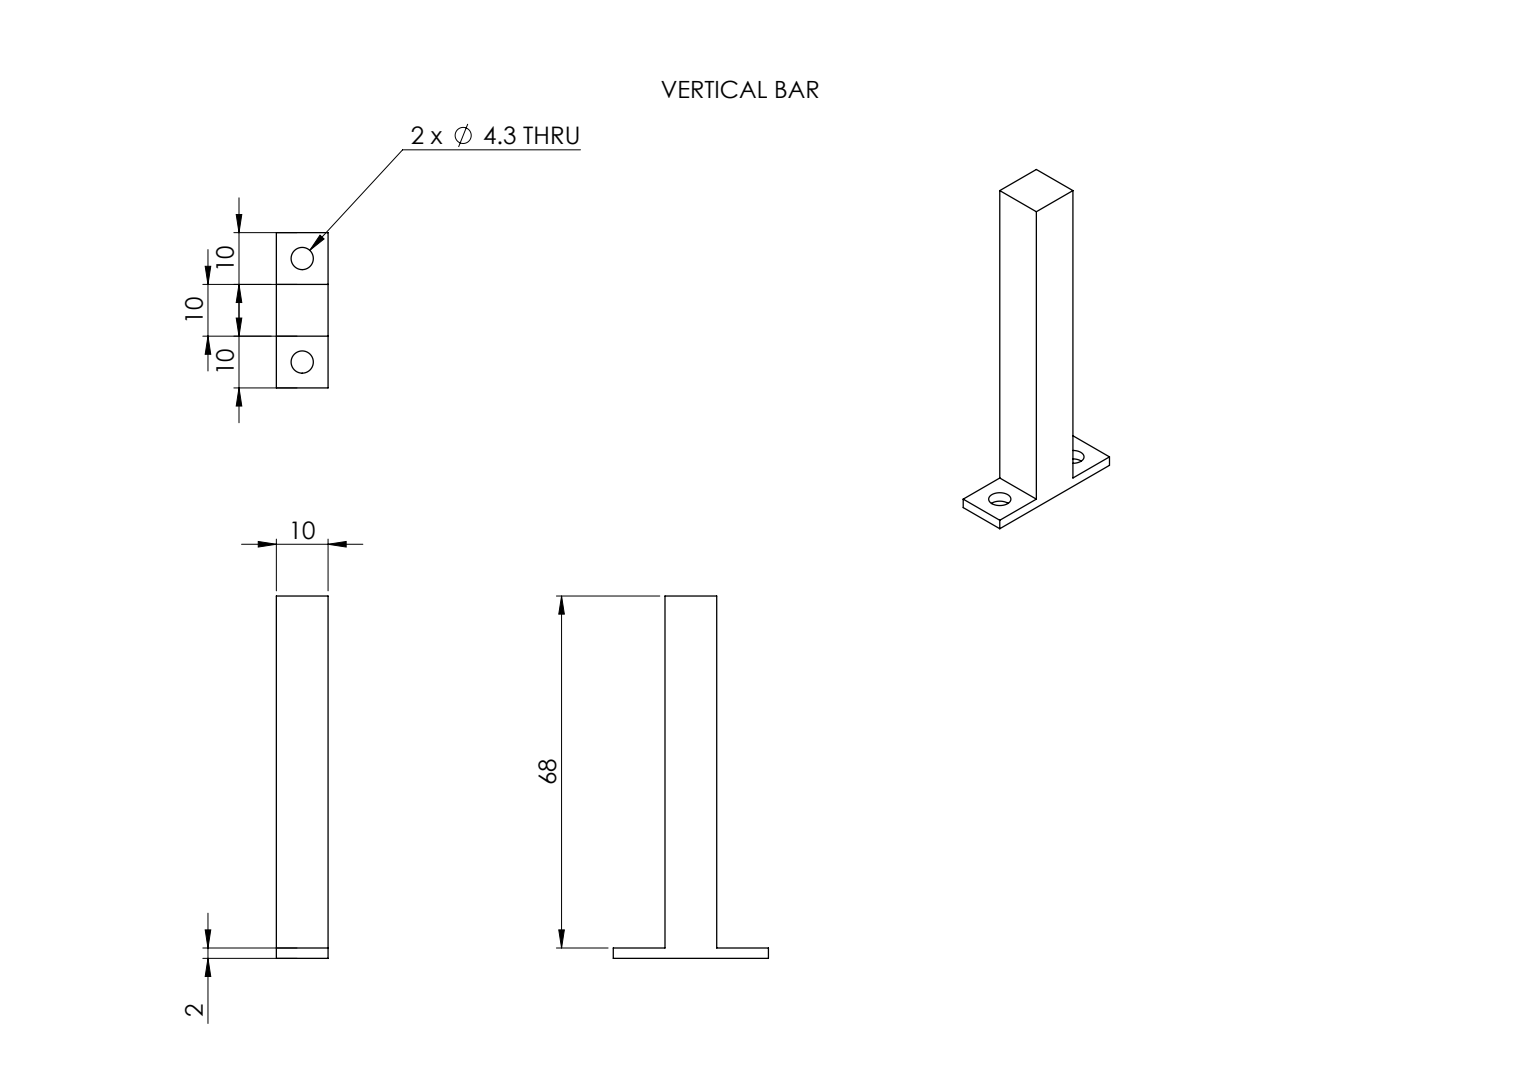
ISO-10303-21;
HEADER;
FILE_DESCRIPTION (('STEP AP214'),
    '1' );
FILE_NAME ('vertical bar^MAS-192.step',
    '2026-10-24T04:45:50',
    ( '' ),
    ( '' ),
    'SwSTEP 2.0',
    'SolidWorks 2026',
    '' );
FILE_SCHEMA (( 'AUTOMOTIVE_DESIGN' ));
ENDSEC;

DATA;
#7=( GEOMETRIC_REPRESENTATION_CONTEXT ( 3 ) GLOBAL_UNCERTAINTY_ASSIGNED_CONTEXT ( ( #487 ) ) GLOBAL_UNIT_ASSIGNED_CONTEXT ( ( #3000, #1213, #165 ) ) REPRESENTATION_CONTEXT ( 'NONE', 'WORKASPACE' ) );
#18=CARTESIAN_POINT ( 'NONE',  ( -49.99999999999999289, 52.00000000000000711, -14.99999999999999645 ) ) ;
#30=CARTESIAN_POINT ( 'NONE',  ( -45.00000000000000000, 52.00000000000000711, -7.849999999999996092 ) ) ;
#40=AXIS2_PLACEMENT_3D ( 'NONE', #1566, #1549, #2083 ) ;
#49=AXIS2_PLACEMENT_3D ( 'NONE', #2635, #3135, #2647 ) ;
#59=VECTOR ( 'NONE', #1910, 1000.000000000000000 ) ;
#68=DIRECTION ( 'NONE',  ( -1.000000000000000000, -0.000000000000000000, -0.000000000000000000 ) ) ;
#69=CARTESIAN_POINT ( 'NONE',  ( -45.00000000000000000, 52.00000000000000711, -9.999999999999994671 ) ) ;
#91=ORIENTED_EDGE ( 'NONE', *, *, #1822, .T. ) ;
#99=DIRECTION ( 'NONE',  ( 0.000000000000000000, -1.000000000000000000, -0.000000000000000000 ) ) ;
#130=LINE ( 'NONE', #2502, #3267 ) ;
#137=EDGE_CURVE ( 'NONE', #1848, #2577, #1400, .T. ) ;
#143=CARTESIAN_POINT ( 'NONE',  ( -49.99999999999998579, 50.00000000000000000, 15.00000000000000888 ) ) ;
#165=( NAMED_UNIT ( * ) SI_UNIT ( $, .STERADIAN. ) SOLID_ANGLE_UNIT ( ) );
#174=CARTESIAN_POINT ( 'NONE',  ( -44.99999999999999289, 52.00000000000000711, 10.00000000000000533 ) ) ;
#177=ADVANCED_FACE ( 'NONE', ( #782 ), #2573, .F. ) ;
#181=EDGE_CURVE ( 'NONE', #2222, #1240, #233, .T. ) ;
#189=DIRECTION ( 'NONE',  ( 0.000000000000000000, 0.000000000000000000, 1.000000000000000000 ) ) ;
#190=VERTEX_POINT ( 'NONE', #1045 ) ;
#194=CARTESIAN_POINT ( 'NONE',  ( -49.99999999999999289, 52.00000000000000711, -4.999999999999995559 ) ) ;
#197=DIRECTION ( 'NONE',  ( -0.000000000000000000, 1.000000000000000000, -0.000000000000000000 ) ) ;
#198=CARTESIAN_POINT ( 'NONE',  ( -50.00000000000000000, 120.0000000000000142, 5.000000000000004441 ) ) ;
#214=ORIENTED_EDGE ( 'NONE', *, *, #2529, .F. ) ;
#217=CARTESIAN_POINT ( 'NONE',  ( -45.00000000000000000, 50.00000000000000000, -9.999999999999994671 ) ) ;
#224=ORIENTED_EDGE ( 'NONE', *, *, #1328, .F. ) ;
#229=VERTEX_POINT ( 'NONE', #2063 ) ;
#233=LINE ( 'NONE', #18, #635 ) ;
#235=PRODUCT ( 'vertical bar^MAS-192', 'vertical bar^MAS-192', '', ( #1405 ) ) ;
#239=DIRECTION ( 'NONE',  ( 1.000000000000000000, 0.000000000000000000, 0.000000000000000000 ) ) ;
#256=PLANE ( 'NONE',  #3270 ) ;
#259=EDGE_CURVE ( 'NONE', #2577, #1848, #1348, .T. ) ;
#285=ORIENTED_EDGE ( 'NONE', *, *, #1596, .F. ) ;
#299=ORIENTED_EDGE ( 'NONE', *, *, #1600, .T. ) ;
#311=FACE_OUTER_BOUND ( 'NONE', #2869, .T. ) ;
#313=ORIENTED_EDGE ( 'NONE', *, *, #934, .T. ) ;
#315=ADVANCED_BREP_SHAPE_REPRESENTATION ( '', ( #2820, #3111 ), #7 ) ;
#316=LINE ( 'NONE', #2146, #2603 ) ;
#318=CIRCLE ( 'NONE', #2498, 2.149999999999999023 ) ;
#326=ORIENTED_EDGE ( 'NONE', *, *, #789, .T. ) ;
#327=EDGE_LOOP ( 'NONE', ( #1272, #3114, #2142, #1931 ) ) ;
#328=FACE_OUTER_BOUND ( 'NONE', #327, .T. ) ;
#336=DIRECTION ( 'NONE',  ( 6.938893903907228378E-16, 0.000000000000000000, 1.000000000000000000 ) ) ;
#344=CARTESIAN_POINT ( 'NONE',  ( -49.99999999999999289, 52.00000000000000711, -14.99999999999999645 ) ) ;
#353=FACE_OUTER_BOUND ( 'NONE', #793, .T. ) ;
#355=EDGE_LOOP ( 'NONE', ( #2017, #2646, #2374, #1630 ) ) ;
#356=LINE ( 'NONE', #823, #1685 ) ;
#358=ORIENTED_EDGE ( 'NONE', *, *, #750, .T. ) ;
#359=CARTESIAN_POINT ( 'NONE',  ( -44.99999999999999289, 50.00000000000000000, 10.00000000000000533 ) ) ;
#361=VERTEX_POINT ( 'NONE', #3180 ) ;
#373=AXIS2_PLACEMENT_3D ( 'NONE', #3007, #3300, #957 ) ;
#392=EDGE_CURVE ( 'NONE', #2543, #2273, #1858, .T. ) ;
#399=DIRECTION ( 'NONE',  ( -0.000000000000000000, 1.000000000000000000, -0.000000000000000000 ) ) ;
#404=FILL_AREA_STYLE_COLOUR ( '', #874 ) ;
#430=LINE ( 'NONE', #1761, #2389 ) ;
#439=( NAMED_UNIT ( * ) PLANE_ANGLE_UNIT ( ) SI_UNIT ( $, .RADIAN. ) );
#447=( LENGTH_UNIT ( ) NAMED_UNIT ( * ) SI_UNIT ( .MILLI., .METRE. ) );
#449=LINE ( 'NONE', #959, #1301 ) ;
#465=ORIENTED_EDGE ( 'NONE', *, *, #2720, .F. ) ;
#471=DIRECTION ( 'NONE',  ( -0.000000000000000000, 1.000000000000000000, -0.000000000000000000 ) ) ;
#476=ORIENTED_EDGE ( 'NONE', *, *, #2240, .T. ) ;
#481=DIRECTION ( 'NONE',  ( 0.000000000000000000, -0.000000000000000000, -1.000000000000000000 ) ) ;
#487=UNCERTAINTY_MEASURE_WITH_UNIT (LENGTH_MEASURE( 1.000000000000000082E-05 ), #3000, 'distance_accuracy_value', 'NONE');
#491=DIRECTION ( 'NONE',  ( -0.000000000000000000, -1.000000000000000000, -0.000000000000000000 ) ) ;
#493=LINE ( 'NONE', #2046, #2452 ) ;
#496=EDGE_CURVE ( 'NONE', #1994, #2222, #130, .T. ) ;
#500=LINE ( 'NONE', #2579, #1737 ) ;
#517=DIRECTION ( 'NONE',  ( -0.000000000000000000, 1.000000000000000000, -0.000000000000000000 ) ) ;
#524=( NAMED_UNIT ( * ) SI_UNIT ( $, .STERADIAN. ) SOLID_ANGLE_UNIT ( ) );
#526=ORIENTED_EDGE ( 'NONE', *, *, #934, .F. ) ;
#529=VECTOR ( 'NONE', #491, 1000.000000000000000 ) ;
#534=VECTOR ( 'NONE', #1624, 1000.000000000000000 ) ;
#538=ORIENTED_EDGE ( 'NONE', *, *, #496, .F. ) ;
#539=DIRECTION ( 'NONE',  ( 0.000000000000000000, -1.000000000000000000, 0.000000000000000000 ) ) ;
#542=AXIS2_PLACEMENT_3D ( 'NONE', #1565, #1586, #1044 ) ;
#558=DIRECTION ( 'NONE',  ( -1.000000000000000000, 0.000000000000000000, 6.938893903907232322E-16 ) ) ;
#574=DIRECTION ( 'NONE',  ( 0.000000000000000000, 0.000000000000000000, 1.000000000000000000 ) ) ;
#580=CARTESIAN_POINT ( 'NONE',  ( -45.00000000000000000, 50.00000000000000000, -7.849999999999996092 ) ) ;
#585=CARTESIAN_POINT ( 'NONE',  ( -44.99999999999999289, 50.00000000000000000, 10.00000000000000533 ) ) ;
#608=VERTEX_POINT ( 'NONE', #2329 ) ;
#610=DIRECTION ( 'NONE',  ( 6.938893903907228378E-16, 0.000000000000000000, -1.000000000000000000 ) ) ;
#614=PLANE ( 'NONE',  #3101 ) ;
#619=EDGE_CURVE ( 'NONE', #1240, #2273, #742, .T. ) ;
#624=VERTEX_POINT ( 'NONE', #2550 ) ;
#635=VECTOR ( 'NONE', #1006, 1000.000000000000000 ) ;
#643=VECTOR ( 'NONE', #2325, 1000.000000000000000 ) ;
#652=LINE ( 'NONE', #1697, #534 ) ;
#667=ORIENTED_EDGE ( 'NONE', *, *, #2408, .F. ) ;
#677=PLANE ( 'NONE',  #2180 ) ;
#682=ORIENTED_EDGE ( 'NONE', *, *, #392, .F. ) ;
#688=DIRECTION ( 'NONE',  ( -0.000000000000000000, 1.000000000000000000, -0.000000000000000000 ) ) ;
#692=ORIENTED_EDGE ( 'NONE', *, *, #3311, .F. ) ;
#699=VERTEX_POINT ( 'NONE', #2973 ) ;
#706=CARTESIAN_POINT ( 'NONE',  ( -49.99999999999998579, 52.00000000000000711, 15.00000000000000888 ) ) ;
#707=SURFACE_SIDE_STYLE ('',( #2258 ) ) ;
#714=SHAPE_REPRESENTATION ( 'vertical bar^MAS-192', ( #3111 ), #7 ) ;
#724=CARTESIAN_POINT ( 'NONE',  ( -45.00000000000000000, 52.00000000000000711, -12.14999999999999503 ) ) ;
#732=EDGE_LOOP ( 'NONE', ( #224, #1699, #2690, #1975 ) ) ;
#740=VERTEX_POINT ( 'NONE', #1944 ) ;
#742=LINE ( 'NONE', #3123, #3097 ) ;
#749=VECTOR ( 'NONE', #1269, 1000.000000000000000 ) ;
#750=EDGE_CURVE ( 'NONE', #624, #1751, #318, .T. ) ;
#759=CARTESIAN_POINT ( 'NONE',  ( -39.99999999999999289, 52.00000000000000711, 15.00000000000000178 ) ) ;
#765=CIRCLE ( 'NONE', #2232, 2.149999999999999023 ) ;
#766=LINE ( 'NONE', #1547, #529 ) ;
#782=FACE_OUTER_BOUND ( 'NONE', #1028, .T. ) ;
#787=VERTEX_POINT ( 'NONE', #580 ) ;
#789=EDGE_CURVE ( 'NONE', #2683, #2543, #652, .T. ) ;
#793=EDGE_LOOP ( 'NONE', ( #299, #2023, #2312, #285 ) ) ;
#796=FACE_BOUND ( 'NONE', #1865, .T. ) ;
#800=ORIENTED_EDGE ( 'NONE', *, *, #1328, .T. ) ;
#810=VECTOR ( 'NONE', #1384, 1000.000000000000000 ) ;
#823=CARTESIAN_POINT ( 'NONE',  ( -40.00000000000000000, 120.0000000000000142, 5.000000000000004441 ) ) ;
#836=CARTESIAN_POINT ( 'NONE',  ( -39.99999999999999289, 52.00000000000000711, 15.00000000000000178 ) ) ;
#845=PLANE ( 'NONE',  #2875 ) ;
#855=ADVANCED_FACE ( 'NONE', ( #1918 ), #614, .F. ) ;
#856=ORIENTED_EDGE ( 'NONE', *, *, #1712, .T. ) ;
#862=DIRECTION ( 'NONE',  ( 0.000000000000000000, -1.000000000000000000, 0.000000000000000000 ) ) ;
#866=CARTESIAN_POINT ( 'NONE',  ( -49.99999999999999289, 120.0000000000000142, -4.999999999999995559 ) ) ;
#869=CARTESIAN_POINT ( 'NONE',  ( -40.00000000000000000, 120.0000000000000142, -4.999999999999995559 ) ) ;
#874=COLOUR_RGB ( '',0.8941176470588234615, 0.8941176470588234615, 0.8941176470588234615 ) ;
#881=LINE ( 'NONE', #3259, #1625 ) ;
#896=DIRECTION ( 'NONE',  ( 0.000000000000000000, 0.000000000000000000, -1.000000000000000000 ) ) ;
#897=( LENGTH_UNIT ( ) NAMED_UNIT ( * ) SI_UNIT ( .MILLI., .METRE. ) );
#922=AXIS2_PLACEMENT_3D ( 'NONE', #1606, #2937, #610 ) ;
#927=ORIENTED_EDGE ( 'NONE', *, *, #2482, .T. ) ;
#934=EDGE_CURVE ( 'NONE', #1751, #1843, #449, .T. ) ;
#941=CARTESIAN_POINT ( 'NONE',  ( -40.00000000000000000, 52.00000000000000711, -4.999999999999996447 ) ) ;
#949=EDGE_CURVE ( 'NONE', #1041, #608, #430, .T. ) ;
#957=DIRECTION ( 'NONE',  ( 0.000000000000000000, 0.000000000000000000, 1.000000000000000000 ) ) ;
#958=ORIENTED_EDGE ( 'NONE', *, *, #1431, .F. ) ;
#959=CARTESIAN_POINT ( 'NONE',  ( -44.99999999999999289, 52.00000000000000711, 12.15000000000000391 ) ) ;
#971=AXIS2_PLACEMENT_3D ( 'NONE', #585, #862, #1870 ) ;
#983=ADVANCED_FACE ( 'NONE', ( #2525 ), #1725, .F. ) ;
#986=APPLICATION_CONTEXT ( 'automotive_design' ) ;
#990=CARTESIAN_POINT ( 'NONE',  ( -45.00000000000000000, 52.00000000000000711, -9.999999999999994671 ) ) ;
#994=ORIENTED_EDGE ( 'NONE', *, *, #2107, .T. ) ;
#1006=DIRECTION ( 'NONE',  ( -0.000000000000000000, -1.000000000000000000, -0.000000000000000000 ) ) ;
#1017=DIRECTION ( 'NONE',  ( -6.938893903907228378E-16, -0.000000000000000000, 1.000000000000000000 ) ) ;
#1020=DIRECTION ( 'NONE',  ( 0.000000000000000000, 0.000000000000000000, 1.000000000000000000 ) ) ;
#1022=LINE ( 'NONE', #2356, #1097 ) ;
#1024=LINE ( 'NONE', #1569, #2229 ) ;
#1028=EDGE_LOOP ( 'NONE', ( #1469, #2196, #1120, #2571 ) ) ;
#1037=LINE ( 'NONE', #724, #1684 ) ;
#1041=VERTEX_POINT ( 'NONE', #2814 ) ;
#1044=DIRECTION ( 'NONE',  ( -1.000000000000000000, 0.000000000000000000, -0.000000000000000000 ) ) ;
#1045=CARTESIAN_POINT ( 'NONE',  ( -45.00000000000000000, 50.00000000000000000, -12.14999999999999503 ) ) ;
#1057=ORIENTED_EDGE ( 'NONE', *, *, #2408, .T. ) ;
#1062=CARTESIAN_POINT ( 'NONE',  ( -50.00000000000000000, 120.0000000000000142, 5.000000000000004441 ) ) ;
#1063=ADVANCED_FACE ( 'NONE', ( #2051, #2102, #3091 ), #256, .T. ) ;
#1064=ORIENTED_EDGE ( 'NONE', *, *, #137, .T. ) ;
#1066=CARTESIAN_POINT ( 'NONE',  ( 0.000000000000000000, 50.00000000000000000, 0.000000000000000000 ) ) ;
#1089=CARTESIAN_POINT ( 'NONE',  ( -45.00000000000000000, 52.00000000000000711, -12.14999999999999503 ) ) ;
#1097=VECTOR ( 'NONE', #1788, 1000.000000000000000 ) ;
#1098=VECTOR ( 'NONE', #471, 1000.000000000000000 ) ;
#1111=EDGE_CURVE ( 'NONE', #1240, #1126, #500, .T. ) ;
#1120=ORIENTED_EDGE ( 'NONE', *, *, #1987, .F. ) ;
#1122=FACE_OUTER_BOUND ( 'NONE', #1948, .T. ) ;
#1123=CARTESIAN_POINT ( 'NONE',  ( -39.99999999999999289, 52.00000000000000711, 15.00000000000000178 ) ) ;
#1126=VERTEX_POINT ( 'NONE', #1812 ) ;
#1144=ADVANCED_FACE ( 'NONE', ( #1657 ), #2918, .F. ) ;
#1148=AXIS2_PLACEMENT_3D ( 'NONE', #836, #1891, #2662 ) ;
#1163=CARTESIAN_POINT ( 'NONE',  ( -45.00000000000000000, 50.00000000000000000, -9.999999999999994671 ) ) ;
#1181=CARTESIAN_POINT ( 'NONE',  ( -40.00000000000000000, 50.00000000000000000, 5.000000000000004441 ) ) ;
#1182=EDGE_CURVE ( 'NONE', #1041, #2643, #356, .T. ) ;
#1185=DIRECTION ( 'NONE',  ( -1.000000000000000000, 0.000000000000000000, 0.000000000000000000 ) ) ;
#1202=CYLINDRICAL_SURFACE ( 'NONE', #373, 2.149999999999999023 ) ;
#1211=EDGE_CURVE ( 'NONE', #787, #190, #765, .T. ) ;
#1213=( NAMED_UNIT ( * ) PLANE_ANGLE_UNIT ( ) SI_UNIT ( $, .RADIAN. ) );
#1240=VERTEX_POINT ( 'NONE', #2645 ) ;
#1249=AXIS2_PLACEMENT_3D ( 'NONE', #174, #2762, #189 ) ;
#1253=VECTOR ( 'NONE', #2781, 1000.000000000000000 ) ;
#1254=ORIENTED_EDGE ( 'NONE', *, *, #2848, .F. ) ;
#1261=ADVANCED_FACE ( 'NONE', ( #1122 ), #3186, .T. ) ;
#1267=DIRECTION ( 'NONE',  ( -0.000000000000000000, -1.000000000000000000, -0.000000000000000000 ) ) ;
#1269=DIRECTION ( 'NONE',  ( -1.000000000000000000, 0.000000000000000000, 0.000000000000000000 ) ) ;
#1271=ADVANCED_FACE ( 'NONE', ( #328 ), #1368, .T. ) ;
#1272=ORIENTED_EDGE ( 'NONE', *, *, #1111, .F. ) ;
#1284=ORIENTED_EDGE ( 'NONE', *, *, #1600, .F. ) ;
#1290=ORIENTED_EDGE ( 'NONE', *, *, #750, .F. ) ;
#1298=ORIENTED_EDGE ( 'NONE', *, *, #3357, .T. ) ;
#1301=VECTOR ( 'NONE', #399, 1000.000000000000000 ) ;
#1315=PLANE ( 'NONE',  #542 ) ;
#1318=DIRECTION ( 'NONE',  ( -0.000000000000000000, -1.000000000000000000, -0.000000000000000000 ) ) ;
#1323=ORIENTED_EDGE ( 'NONE', *, *, #1607, .F. ) ;
#1328=EDGE_CURVE ( 'NONE', #2543, #1126, #2741, .T. ) ;
#1329=FACE_OUTER_BOUND ( 'NONE', #1663, .T. ) ;
#1348=CIRCLE ( 'NONE', #1892, 2.149999999999999023 ) ;
#1355=VECTOR ( 'NONE', #1530, 1000.000000000000000 ) ;
#1365=ORIENTED_EDGE ( 'NONE', *, *, #1211, .F. ) ;
#1368=PLANE ( 'NONE',  #2826 ) ;
#1380=PLANE ( 'NONE',  #1687 ) ;
#1383=DIRECTION ( 'NONE',  ( 0.000000000000000000, 0.000000000000000000, -1.000000000000000000 ) ) ;
#1384=DIRECTION ( 'NONE',  ( 1.000000000000000000, 0.000000000000000000, 0.000000000000000000 ) ) ;
#1400=CIRCLE ( 'NONE', #3092, 2.149999999999999023 ) ;
#1402=DIRECTION ( 'NONE',  ( 0.000000000000000000, 0.000000000000000000, -1.000000000000000000 ) ) ;
#1405=PRODUCT_CONTEXT ( 'NONE', #986, 'mechanical' ) ;
#1424=ORIENTED_EDGE ( 'NONE', *, *, #1987, .T. ) ;
#1431=EDGE_CURVE ( 'NONE', #2174, #3236, #3284, .T. ) ;
#1440=FILL_AREA_STYLE ('',( #404 ) ) ;
#1442=CARTESIAN_POINT ( 'NONE',  ( -44.99999999999999289, 52.00000000000000711, 10.00000000000000533 ) ) ;
#1444=ADVANCED_FACE ( 'NONE', ( #3020 ), #677, .F. ) ;
#1469=ORIENTED_EDGE ( 'NONE', *, *, #3129, .T. ) ;
#1475=ORIENTED_EDGE ( 'NONE', *, *, #3129, .F. ) ;
#1480=DIRECTION ( 'NONE',  ( 0.000000000000000000, 0.000000000000000000, 1.000000000000000000 ) ) ;
#1486=ORIENTED_EDGE ( 'NONE', *, *, #1804, .T. ) ;
#1511=AXIS2_PLACEMENT_3D ( 'NONE', #1442, #688, #1480 ) ;
#1518=FACE_OUTER_BOUND ( 'NONE', #2894, .T. ) ;
#1530=DIRECTION ( 'NONE',  ( -1.000000000000000000, 0.000000000000000000, 6.938893903907232322E-16 ) ) ;
#1531=VERTEX_POINT ( 'NONE', #1062 ) ;
#1542=ORIENTED_EDGE ( 'NONE', *, *, #2186, .T. ) ;
#1545=ORIENTED_EDGE ( 'NONE', *, *, #1804, .F. ) ;
#1547=CARTESIAN_POINT ( 'NONE',  ( -49.99999999999999289, 120.0000000000000142, -4.999999999999995559 ) ) ;
#1549=DIRECTION ( 'NONE',  ( 0.000000000000000000, 0.000000000000000000, 1.000000000000000000 ) ) ;
#1550=CARTESIAN_POINT ( 'NONE',  ( -40.00000000000000000, 52.00000000000000711, -4.999999999999996447 ) ) ;
#1565=CARTESIAN_POINT ( 'NONE',  ( 0.000000000000000000, 52.00000000000000711, 0.000000000000000000 ) ) ;
#1566=CARTESIAN_POINT ( 'NONE',  ( -49.99999999999999289, 120.0000000000000142, -4.999999999999995559 ) ) ;
#1569=CARTESIAN_POINT ( 'NONE',  ( -40.00000000000000000, 52.00000000000000711, -14.99999999999999645 ) ) ;
#1586=DIRECTION ( 'NONE',  ( 0.000000000000000000, -1.000000000000000000, -0.000000000000000000 ) ) ;
#1595=CYLINDRICAL_SURFACE ( 'NONE', #49, 2.149999999999999023 ) ;
#1596=EDGE_CURVE ( 'NONE', #361, #608, #2608, .T. ) ;
#1600=EDGE_CURVE ( 'NONE', #361, #699, #1022, .T. ) ;
#1604=ORIENTED_EDGE ( 'NONE', *, *, #2037, .F. ) ;
#1606=CARTESIAN_POINT ( 'NONE',  ( -50.00000000000000000, 120.0000000000000142, 5.000000000000004441 ) ) ;
#1607=EDGE_CURVE ( 'NONE', #2174, #1994, #2628, .T. ) ;
#1612=FACE_OUTER_BOUND ( 'NONE', #2099, .T. ) ;
#1621=CARTESIAN_POINT ( 'NONE',  ( -40.00000000000000000, 120.0000000000000142, -4.999999999999995559 ) ) ;
#1624=DIRECTION ( 'NONE',  ( -0.000000000000000000, -1.000000000000000000, -0.000000000000000000 ) ) ;
#1625=VECTOR ( 'NONE', #2256, 1000.000000000000000 ) ;
#1630=ORIENTED_EDGE ( 'NONE', *, *, #2240, .F. ) ;
#1632=( GEOMETRIC_REPRESENTATION_CONTEXT ( 3 ) GLOBAL_UNCERTAINTY_ASSIGNED_CONTEXT ( ( #2944 ) ) GLOBAL_UNIT_ASSIGNED_CONTEXT ( ( #447, #3338, #524 ) ) REPRESENTATION_CONTEXT ( 'NONE', 'WORKASPACE' ) );
#1645=EDGE_LOOP ( 'NONE', ( #667, #2491, #1298, #1064 ) ) ;
#1657=FACE_OUTER_BOUND ( 'NONE', #1862, .T. ) ;
#1659=ORIENTED_EDGE ( 'NONE', *, *, #2417, .T. ) ;
#1660=CARTESIAN_POINT ( 'NONE',  ( -40.00000000000000000, 120.0000000000000142, 5.000000000000004441 ) ) ;
#1663=EDGE_LOOP ( 'NONE', ( #1890, #465, #538, #1323 ) ) ;
#1678=APPLICATION_CONTEXT ( 'automotive_design' ) ;
#1681=CIRCLE ( 'NONE', #1894, 2.149999999999999023 ) ;
#1684=VECTOR ( 'NONE', #517, 1000.000000000000000 ) ;
#1685=VECTOR ( 'NONE', #2140, 1000.000000000000000 ) ;
#1687=AXIS2_PLACEMENT_3D ( 'NONE', #2459, #99, #2967 ) ;
#1697=CARTESIAN_POINT ( 'NONE',  ( -39.99999999999999289, 52.00000000000000711, 15.00000000000000178 ) ) ;
#1699=ORIENTED_EDGE ( 'NONE', *, *, #392, .T. ) ;
#1700=CARTESIAN_POINT ( 'NONE',  ( -49.99999999999999289, 52.00000000000000711, -14.99999999999999645 ) ) ;
#1702=( NAMED_UNIT ( * ) SI_UNIT ( $, .STERADIAN. ) SOLID_ANGLE_UNIT ( ) );
#1710=DIRECTION ( 'NONE',  ( -0.000000000000000000, -1.000000000000000000, -0.000000000000000000 ) ) ;
#1712=EDGE_CURVE ( 'NONE', #2643, #229, #2914, .T. ) ;
#1722=DIRECTION ( 'NONE',  ( 0.000000000000000000, 0.000000000000000000, -1.000000000000000000 ) ) ;
#1725=CYLINDRICAL_SURFACE ( 'NONE', #1249, 2.149999999999999023 ) ;
#1730=PRESENTATION_STYLE_ASSIGNMENT (( #3246 ) ) ;
#1737=VECTOR ( 'NONE', #239, 1000.000000000000000 ) ;
#1745=MECHANICAL_DESIGN_GEOMETRIC_PRESENTATION_REPRESENTATION('',(#2235),#2722);
#1751=VERTEX_POINT ( 'NONE', #2416 ) ;
#1761=CARTESIAN_POINT ( 'NONE',  ( -40.00000000000000000, 120.0000000000000142, 5.000000000000004441 ) ) ;
#1765=LINE ( 'NONE', #759, #1355 ) ;
#1766=ORIENTED_EDGE ( 'NONE', *, *, #3357, .F. ) ;
#1788=DIRECTION ( 'NONE',  ( 6.938893903907228378E-16, 0.000000000000000000, 1.000000000000000000 ) ) ;
#1792=VECTOR ( 'NONE', #1851, 1000.000000000000000 ) ;
#1794=EDGE_LOOP ( 'NONE', ( #800, #1254, #958, #1475, #3271, #1984, #994, #326 ) ) ;
#1804=EDGE_CURVE ( 'NONE', #229, #1531, #1859, .T. ) ;
#1812=CARTESIAN_POINT ( 'NONE',  ( -40.00000000000000000, 50.00000000000000000, -14.99999999999999645 ) ) ;
#1817=ORIENTED_EDGE ( 'NONE', *, *, #181, .T. ) ;
#1822=EDGE_CURVE ( 'NONE', #1843, #740, #2654, .T. ) ;
#1843=VERTEX_POINT ( 'NONE', #2213 ) ;
#1848=VERTEX_POINT ( 'NONE', #2005 ) ;
#1850=VECTOR ( 'NONE', #2641, 1000.000000000000000 ) ;
#1851=DIRECTION ( 'NONE',  ( -0.000000000000000000, 1.000000000000000000, -0.000000000000000000 ) ) ;
#1855=ORIENTED_EDGE ( 'NONE', *, *, #137, .F. ) ;
#1858=LINE ( 'NONE', #2640, #2931 ) ;
#1859=LINE ( 'NONE', #2898, #1850 ) ;
#1862=EDGE_LOOP ( 'NONE', ( #2990, #2526, #1284, #692, #1545, #1424, #3319, #1817 ) ) ;
#1865=EDGE_LOOP ( 'NONE', ( #1855, #2824 ) ) ;
#1866=CARTESIAN_POINT ( 'NONE',  ( -39.99999999999999289, 50.00000000000000000, 15.00000000000000178 ) ) ;
#1870=DIRECTION ( 'NONE',  ( 0.000000000000000000, 0.000000000000000000, -1.000000000000000000 ) ) ;
#1871=CARTESIAN_POINT ( 'NONE',  ( 0.000000000000000000, 0.000000000000000000, 0.000000000000000000 ) ) ;
#1890=ORIENTED_EDGE ( 'NONE', *, *, #1431, .T. ) ;
#1891=DIRECTION ( 'NONE',  ( 6.938893903907232322E-16, -0.000000000000000000, 1.000000000000000000 ) ) ;
#1892=AXIS2_PLACEMENT_3D ( 'NONE', #990, #2031, #2808 ) ;
#1894=AXIS2_PLACEMENT_3D ( 'NONE', #1163, #3245, #896 ) ;
#1910=DIRECTION ( 'NONE',  ( -0.000000000000000000, -1.000000000000000000, -0.000000000000000000 ) ) ;
#1917=EDGE_LOOP ( 'NONE', ( #1365, #2615 ) ) ;
#1918=FACE_OUTER_BOUND ( 'NONE', #1794, .T. ) ;
#1920=ORIENTED_EDGE ( 'NONE', *, *, #259, .T. ) ;
#1931=ORIENTED_EDGE ( 'NONE', *, *, #2848, .T. ) ;
#1944=CARTESIAN_POINT ( 'NONE',  ( -44.99999999999999289, 52.00000000000000711, 7.850000000000005862 ) ) ;
#1948=EDGE_LOOP ( 'NONE', ( #682, #2323, #1659, #927 ) ) ;
#1975=ORIENTED_EDGE ( 'NONE', *, *, #1111, .T. ) ;
#1980=DIRECTION ( 'NONE',  ( 0.000000000000000000, 0.000000000000000000, 1.000000000000000000 ) ) ;
#1984=ORIENTED_EDGE ( 'NONE', *, *, #949, .T. ) ;
#1987=EDGE_CURVE ( 'NONE', #229, #1994, #766, .T. ) ;
#1994=VERTEX_POINT ( 'NONE', #194 ) ;
#2005=CARTESIAN_POINT ( 'NONE',  ( -45.00000000000000000, 52.00000000000000711, -7.849999999999996092 ) ) ;
#2009=STYLED_ITEM('',(#3415),#2820);
#2017=ORIENTED_EDGE ( 'NONE', *, *, #3311, .T. ) ;
#2023=ORIENTED_EDGE ( 'NONE', *, *, #2417, .F. ) ;
#2031=DIRECTION ( 'NONE',  ( -0.000000000000000000, 1.000000000000000000, -0.000000000000000000 ) ) ;
#2037=EDGE_CURVE ( 'NONE', #740, #1843, #2171, .T. ) ;
#2046=CARTESIAN_POINT ( 'NONE',  ( -50.00000000000000000, 120.0000000000000142, 5.000000000000004441 ) ) ;
#2048=DIRECTION ( 'NONE',  ( 1.000000000000000000, 0.000000000000000000, -6.938893903907232322E-16 ) ) ;
#2051=FACE_BOUND ( 'NONE', #1917, .T. ) ;
#2063=CARTESIAN_POINT ( 'NONE',  ( -49.99999999999999289, 120.0000000000000142, -4.999999999999995559 ) ) ;
#2076=ORIENTED_EDGE ( 'NONE', *, *, #2037, .T. ) ;
#2083=DIRECTION ( 'NONE',  ( 1.000000000000000000, 0.000000000000000000, -0.000000000000000000 ) ) ;
#2099=EDGE_LOOP ( 'NONE', ( #3068, #856, #1486, #476 ) ) ;
#2102=FACE_BOUND ( 'NONE', #3090, .T. ) ;
#2107=EDGE_CURVE ( 'NONE', #608, #2683, #316, .T. ) ;
#2122=ADVANCED_FACE ( 'NONE', ( #1612 ), #845, .F. ) ;
#2140=DIRECTION ( 'NONE',  ( 0.000000000000000000, 0.000000000000000000, -1.000000000000000000 ) ) ;
#2142=ORIENTED_EDGE ( 'NONE', *, *, #2720, .T. ) ;
#2146=CARTESIAN_POINT ( 'NONE',  ( -40.00000000000000000, 52.00000000000000711, 5.000000000000000888 ) ) ;
#2153=DIRECTION ( 'NONE',  ( -1.000000000000000000, 0.000000000000000000, -0.000000000000000000 ) ) ;
#2165=DIRECTION ( 'NONE',  ( -0.000000000000000000, 1.000000000000000000, -0.000000000000000000 ) ) ;
#2171=CIRCLE ( 'NONE', #2658, 2.149999999999999023 ) ;
#2174=VERTEX_POINT ( 'NONE', #2182 ) ;
#2180=AXIS2_PLACEMENT_3D ( 'NONE', #198, #1722, #2757 ) ;
#2182=CARTESIAN_POINT ( 'NONE',  ( -40.00000000000000000, 52.00000000000000711, -4.999999999999996447 ) ) ;
#2186=EDGE_CURVE ( 'NONE', #1751, #624, #2547, .T. ) ;
#2188=EDGE_LOOP ( 'NONE', ( #2310, #1604 ) ) ;
#2195=SHAPE_DEFINITION_REPRESENTATION ( #3103, #714 ) ;
#2196=ORIENTED_EDGE ( 'NONE', *, *, #1607, .T. ) ;
#2207=DIRECTION ( 'NONE',  ( 0.000000000000000000, -1.000000000000000000, 0.000000000000000000 ) ) ;
#2213=CARTESIAN_POINT ( 'NONE',  ( -44.99999999999999289, 52.00000000000000711, 12.15000000000000391 ) ) ;
#2222=VERTEX_POINT ( 'NONE', #1700 ) ;
#2229=VECTOR ( 'NONE', #1318, 1000.000000000000000 ) ;
#2232=AXIS2_PLACEMENT_3D ( 'NONE', #217, #2332, #2555 ) ;
#2235=STYLED_ITEM ( 'NONE', ( #1730 ), #315 ) ;
#2240=EDGE_CURVE ( 'NONE', #1531, #1041, #881, .T. ) ;
#2256=DIRECTION ( 'NONE',  ( 1.000000000000000000, 0.000000000000000000, 0.000000000000000000 ) ) ;
#2258=SURFACE_STYLE_FILL_AREA ( #1440 ) ;
#2273=VERTEX_POINT ( 'NONE', #143 ) ;
#2279=DIRECTION ( 'NONE',  ( 0.000000000000000000, 0.000000000000000000, 1.000000000000000000 ) ) ;
#2284=VECTOR ( 'NONE', #2048, 1000.000000000000000 ) ;
#2299=DIRECTION ( 'NONE',  ( -0.000000000000000000, 1.000000000000000000, -0.000000000000000000 ) ) ;
#2300=LINE ( 'NONE', #30, #1098 ) ;
#2310=ORIENTED_EDGE ( 'NONE', *, *, #1822, .F. ) ;
#2312=ORIENTED_EDGE ( 'NONE', *, *, #2107, .F. ) ;
#2323=ORIENTED_EDGE ( 'NONE', *, *, #789, .F. ) ;
#2325=DIRECTION ( 'NONE',  ( -0.000000000000000000, -1.000000000000000000, -0.000000000000000000 ) ) ;
#2329=CARTESIAN_POINT ( 'NONE',  ( -40.00000000000000000, 52.00000000000000711, 5.000000000000004441 ) ) ;
#2332=DIRECTION ( 'NONE',  ( 0.000000000000000000, -1.000000000000000000, 0.000000000000000000 ) ) ;
#2334=EDGE_CURVE ( 'NONE', #190, #787, #1681, .T. ) ;
#2356=CARTESIAN_POINT ( 'NONE',  ( -49.99999999999999289, 52.00000000000000711, 5.000000000000007994 ) ) ;
#2374=ORIENTED_EDGE ( 'NONE', *, *, #949, .F. ) ;
#2379=LINE ( 'NONE', #2870, #1792 ) ;
#2381=DIRECTION ( 'NONE',  ( 0.000000000000000000, -0.000000000000000000, -1.000000000000000000 ) ) ;
#2386=CYLINDRICAL_SURFACE ( 'NONE', #3172, 2.149999999999999023 ) ;
#2389=VECTOR ( 'NONE', #1710, 1000.000000000000000 ) ;
#2404=FACE_OUTER_BOUND ( 'NONE', #1645, .T. ) ;
#2407=CARTESIAN_POINT ( 'NONE',  ( -49.99999999999999289, 52.00000000000000711, -14.99999999999999645 ) ) ;
#2408=EDGE_CURVE ( 'NONE', #190, #2577, #1037, .T. ) ;
#2416=CARTESIAN_POINT ( 'NONE',  ( -44.99999999999999289, 50.00000000000000000, 12.15000000000000391 ) ) ;
#2417=EDGE_CURVE ( 'NONE', #2683, #699, #1765, .T. ) ;
#2429=CARTESIAN_POINT ( 'NONE',  ( 0.000000000000000000, 120.0000000000000142, 0.000000000000000000 ) ) ;
#2452=VECTOR ( 'NONE', #1267, 1000.000000000000000 ) ;
#2459=CARTESIAN_POINT ( 'NONE',  ( 0.000000000000000000, 52.00000000000000711, 0.000000000000000000 ) ) ;
#2466=PRODUCT_DEFINITION_CONTEXT ( 'detailed design', #1678, 'design' ) ;
#2482=EDGE_CURVE ( 'NONE', #699, #2273, #3096, .T. ) ;
#2491=ORIENTED_EDGE ( 'NONE', *, *, #2334, .T. ) ;
#2498=AXIS2_PLACEMENT_3D ( 'NONE', #359, #2207, #1402 ) ;
#2502=CARTESIAN_POINT ( 'NONE',  ( -49.99999999999999289, 52.00000000000000711, -4.999999999999996447 ) ) ;
#2525=FACE_OUTER_BOUND ( 'NONE', #2563, .T. ) ;
#2526=ORIENTED_EDGE ( 'NONE', *, *, #2482, .F. ) ;
#2529=EDGE_CURVE ( 'NONE', #624, #740, #2379, .T. ) ;
#2543=VERTEX_POINT ( 'NONE', #1866 ) ;
#2547=CIRCLE ( 'NONE', #971, 2.149999999999999023 ) ;
#2550=CARTESIAN_POINT ( 'NONE',  ( -44.99999999999999289, 50.00000000000000000, 7.850000000000005862 ) ) ;
#2555=DIRECTION ( 'NONE',  ( 0.000000000000000000, 0.000000000000000000, -1.000000000000000000 ) ) ;
#2563=EDGE_LOOP ( 'NONE', ( #214, #358, #313, #91 ) ) ;
#2569=ADVANCED_FACE ( 'NONE', ( #311 ), #1595, .F. ) ;
#2571=ORIENTED_EDGE ( 'NONE', *, *, #1712, .F. ) ;
#2573=PLANE ( 'NONE',  #40 ) ;
#2577=VERTEX_POINT ( 'NONE', #1089 ) ;
#2579=CARTESIAN_POINT ( 'NONE',  ( -49.99999999999999289, 50.00000000000000000, -14.99999999999999645 ) ) ;
#2603=VECTOR ( 'NONE', #336, 1000.000000000000000 ) ;
#2608=LINE ( 'NONE', #3366, #2284 ) ;
#2615=ORIENTED_EDGE ( 'NONE', *, *, #2334, .F. ) ;
#2628=LINE ( 'NONE', #1550, #749 ) ;
#2635=CARTESIAN_POINT ( 'NONE',  ( -44.99999999999999289, 52.00000000000000711, 10.00000000000000533 ) ) ;
#2639=DIRECTION ( 'NONE',  ( 1.000000000000000000, 0.000000000000000000, 0.000000000000000000 ) ) ;
#2640=CARTESIAN_POINT ( 'NONE',  ( -39.99999999999999289, 50.00000000000000000, 15.00000000000000178 ) ) ;
#2641=DIRECTION ( 'NONE',  ( -6.938893903907228378E-16, -0.000000000000000000, 1.000000000000000000 ) ) ;
#2643=VERTEX_POINT ( 'NONE', #1621 ) ;
#2645=CARTESIAN_POINT ( 'NONE',  ( -49.99999999999999289, 50.00000000000000000, -14.99999999999999645 ) ) ;
#2646=ORIENTED_EDGE ( 'NONE', *, *, #1596, .T. ) ;
#2647=DIRECTION ( 'NONE',  ( 0.000000000000000000, 0.000000000000000000, 1.000000000000000000 ) ) ;
#2654=CIRCLE ( 'NONE', #1511, 2.149999999999999023 ) ;
#2658=AXIS2_PLACEMENT_3D ( 'NONE', #3104, #2299, #2279 ) ;
#2662=DIRECTION ( 'NONE',  ( 1.000000000000000000, 0.000000000000000000, -6.938893903907232322E-16 ) ) ;
#2680=LINE ( 'NONE', #344, #810 ) ;
#2683=VERTEX_POINT ( 'NONE', #1123 ) ;
#2690=ORIENTED_EDGE ( 'NONE', *, *, #619, .F. ) ;
#2714=VECTOR ( 'NONE', #2729, 1000.000000000000000 ) ;
#2720=EDGE_CURVE ( 'NONE', #2222, #3236, #2680, .T. ) ;
#2722=( GEOMETRIC_REPRESENTATION_CONTEXT ( 3 ) GLOBAL_UNCERTAINTY_ASSIGNED_CONTEXT ( ( #3120 ) ) GLOBAL_UNIT_ASSIGNED_CONTEXT ( ( #897, #439, #1702 ) ) REPRESENTATION_CONTEXT ( 'NONE', 'WORKASPACE' ) );
#2729=DIRECTION ( 'NONE',  ( 0.000000000000000000, 0.000000000000000000, -1.000000000000000000 ) ) ;
#2741=LINE ( 'NONE', #1181, #2714 ) ;
#2757=DIRECTION ( 'NONE',  ( -1.000000000000000000, 0.000000000000000000, -0.000000000000000000 ) ) ;
#2759=ADVANCED_FACE ( 'NONE', ( #1518 ), #1202, .F. ) ;
#2762=DIRECTION ( 'NONE',  ( -0.000000000000000000, 1.000000000000000000, -0.000000000000000000 ) ) ;
#2781=DIRECTION ( 'NONE',  ( 0.000000000000000000, 0.000000000000000000, -1.000000000000000000 ) ) ;
#2808=DIRECTION ( 'NONE',  ( 0.000000000000000000, 0.000000000000000000, 1.000000000000000000 ) ) ;
#2814=CARTESIAN_POINT ( 'NONE',  ( -40.00000000000000000, 120.0000000000000142, 5.000000000000004441 ) ) ;
#2820=MANIFOLD_SOLID_BREP ( 'M4 Clearance Hole1', #3367 ) ;
#2824=ORIENTED_EDGE ( 'NONE', *, *, #259, .F. ) ;
#2826=AXIS2_PLACEMENT_3D ( 'NONE', #2407, #1383, #2153 ) ;
#2838=PRODUCT_DEFINITION_FORMATION_WITH_SPECIFIED_SOURCE ( 'ANY', '', #235, .NOT_KNOWN. ) ;
#2848=EDGE_CURVE ( 'NONE', #3236, #1126, #1024, .T. ) ;
#2869=EDGE_LOOP ( 'NONE', ( #1542, #3037, #2076, #526 ) ) ;
#2870=CARTESIAN_POINT ( 'NONE',  ( -44.99999999999999289, 52.00000000000000711, 7.850000000000005862 ) ) ;
#2875=AXIS2_PLACEMENT_3D ( 'NONE', #2429, #539, #2381 ) ;
#2894=EDGE_LOOP ( 'NONE', ( #3343, #1057, #1920, #1766 ) ) ;
#2898=CARTESIAN_POINT ( 'NONE',  ( -50.00000000000000000, 120.0000000000000142, 5.000000000000004441 ) ) ;
#2914=LINE ( 'NONE', #866, #2995 ) ;
#2918=PLANE ( 'NONE',  #922 ) ;
#2931=VECTOR ( 'NONE', #558, 1000.000000000000000 ) ;
#2937=DIRECTION ( 'NONE',  ( 1.000000000000000000, -0.000000000000000000, 6.938893903907228378E-16 ) ) ;
#2944=UNCERTAINTY_MEASURE_WITH_UNIT (LENGTH_MEASURE( 1.000000000000000082E-05 ), #447, 'distance_accuracy_value', 'NONE');
#2967=DIRECTION ( 'NONE',  ( -1.000000000000000000, 0.000000000000000000, -0.000000000000000000 ) ) ;
#2973=CARTESIAN_POINT ( 'NONE',  ( -49.99999999999998579, 52.00000000000000711, 15.00000000000000888 ) ) ;
#2974=ADVANCED_FACE ( 'NONE', ( #3249, #353 ), #1380, .F. ) ;
#2978=DIRECTION ( 'NONE',  ( 0.000000000000000000, 0.000000000000000000, -1.000000000000000000 ) ) ;
#2980=PRODUCT_DEFINITION ( 'UNKNOWN', '', #2838, #2466 ) ;
#2990=ORIENTED_EDGE ( 'NONE', *, *, #619, .T. ) ;
#2995=VECTOR ( 'NONE', #68, 1000.000000000000000 ) ;
#3000=( LENGTH_UNIT ( ) NAMED_UNIT ( * ) SI_UNIT ( .MILLI., .METRE. ) );
#3007=CARTESIAN_POINT ( 'NONE',  ( -45.00000000000000000, 52.00000000000000711, -9.999999999999994671 ) ) ;
#3020=FACE_OUTER_BOUND ( 'NONE', #355, .T. ) ;
#3037=ORIENTED_EDGE ( 'NONE', *, *, #2529, .T. ) ;
#3068=ORIENTED_EDGE ( 'NONE', *, *, #1182, .T. ) ;
#3090=EDGE_LOOP ( 'NONE', ( #3243, #1290 ) ) ;
#3091=FACE_OUTER_BOUND ( 'NONE', #732, .T. ) ;
#3092=AXIS2_PLACEMENT_3D ( 'NONE', #3350, #197, #1020 ) ;
#3096=LINE ( 'NONE', #706, #643 ) ;
#3097=VECTOR ( 'NONE', #1017, 1000.000000000000000 ) ;
#3098=ADVANCED_FACE ( 'NONE', ( #2404 ), #2386, .F. ) ;
#3101=AXIS2_PLACEMENT_3D ( 'NONE', #1660, #1185, #1980 ) ;
#3103=PRODUCT_DEFINITION_SHAPE ( 'NONE', 'NONE',  #2980 ) ;
#3104=CARTESIAN_POINT ( 'NONE',  ( -44.99999999999999289, 52.00000000000000711, 10.00000000000000533 ) ) ;
#3108=MECHANICAL_DESIGN_GEOMETRIC_PRESENTATION_REPRESENTATION('',(#2009),#1632);
#3111=AXIS2_PLACEMENT_3D ( 'NONE', #1871, #3207, #2639 ) ;
#3114=ORIENTED_EDGE ( 'NONE', *, *, #181, .F. ) ;
#3120=UNCERTAINTY_MEASURE_WITH_UNIT (LENGTH_MEASURE( 1.000000000000000082E-05 ), #897, 'distance_accuracy_value', 'NONE');
#3123=CARTESIAN_POINT ( 'NONE',  ( -50.00000000000000000, 50.00000000000000000, 5.000000000000004441 ) ) ;
#3129=EDGE_CURVE ( 'NONE', #2643, #2174, #3214, .T. ) ;
#3135=DIRECTION ( 'NONE',  ( -0.000000000000000000, 1.000000000000000000, -0.000000000000000000 ) ) ;
#3147=DIRECTION ( 'NONE',  ( 0.000000000000000000, -1.000000000000000000, 0.000000000000000000 ) ) ;
#3172=AXIS2_PLACEMENT_3D ( 'NONE', #69, #2165, #574 ) ;
#3180=CARTESIAN_POINT ( 'NONE',  ( -49.99999999999999289, 52.00000000000000711, 5.000000000000007994 ) ) ;
#3186=PLANE ( 'NONE',  #1148 ) ;
#3207=DIRECTION ( 'NONE',  ( 0.000000000000000000, 0.000000000000000000, 1.000000000000000000 ) ) ;
#3214=LINE ( 'NONE', #869, #59 ) ;
#3236=VERTEX_POINT ( 'NONE', #3312 ) ;
#3243=ORIENTED_EDGE ( 'NONE', *, *, #2186, .F. ) ;
#3245=DIRECTION ( 'NONE',  ( 0.000000000000000000, -1.000000000000000000, 0.000000000000000000 ) ) ;
#3246=SURFACE_STYLE_USAGE ( .BOTH. , #707 ) ;
#3249=FACE_BOUND ( 'NONE', #2188, .T. ) ;
#3259=CARTESIAN_POINT ( 'NONE',  ( -50.00000000000000000, 120.0000000000000142, 5.000000000000004441 ) ) ;
#3267=VECTOR ( 'NONE', #2978, 1000.000000000000000 ) ;
#3270=AXIS2_PLACEMENT_3D ( 'NONE', #1066, #3147, #481 ) ;
#3271=ORIENTED_EDGE ( 'NONE', *, *, #1182, .F. ) ;
#3283=ADVANCED_FACE ( 'NONE', ( #796, #1329 ), #1315, .F. ) ;
#3284=LINE ( 'NONE', #941, #1253 ) ;
#3300=DIRECTION ( 'NONE',  ( -0.000000000000000000, 1.000000000000000000, -0.000000000000000000 ) ) ;
#3307=SHAPE_REPRESENTATION_RELATIONSHIP ( 'NONE' , 'NONE' ,  #714, #315 ) ;
#3311=EDGE_CURVE ( 'NONE', #1531, #361, #493, .T. ) ;
#3312=CARTESIAN_POINT ( 'NONE',  ( -40.00000000000000000, 52.00000000000000711, -14.99999999999999645 ) ) ;
#3319=ORIENTED_EDGE ( 'NONE', *, *, #496, .T. ) ;
#3338=( NAMED_UNIT ( * ) PLANE_ANGLE_UNIT ( ) SI_UNIT ( $, .RADIAN. ) );
#3343=ORIENTED_EDGE ( 'NONE', *, *, #1211, .T. ) ;
#3350=CARTESIAN_POINT ( 'NONE',  ( -45.00000000000000000, 52.00000000000000711, -9.999999999999994671 ) ) ;
#3357=EDGE_CURVE ( 'NONE', #787, #1848, #2300, .T. ) ;
#3366=CARTESIAN_POINT ( 'NONE',  ( -49.99999999999999289, 52.00000000000000711, 5.000000000000007994 ) ) ;
#3367=CLOSED_SHELL ( 'NONE', ( #2759, #2569, #855, #177, #1144, #1444, #2122, #1063, #1261, #2974, #1271, #3283, #983, #3098 ) ) ;
#3409=COLOUR_RGB('Grey',0.48,0.52,0.57);
#3410=FILL_AREA_STYLE_COLOUR('',#3409);
#3411=FILL_AREA_STYLE('',(#3410));
#3412=SURFACE_STYLE_FILL_AREA(#3411);
#3413=SURFACE_SIDE_STYLE('',(#3412));
#3414=SURFACE_STYLE_USAGE(.BOTH.,#3413);
#3415=PRESENTATION_STYLE_ASSIGNMENT((#3414));
ENDSEC;
END-ISO-10303-21;
